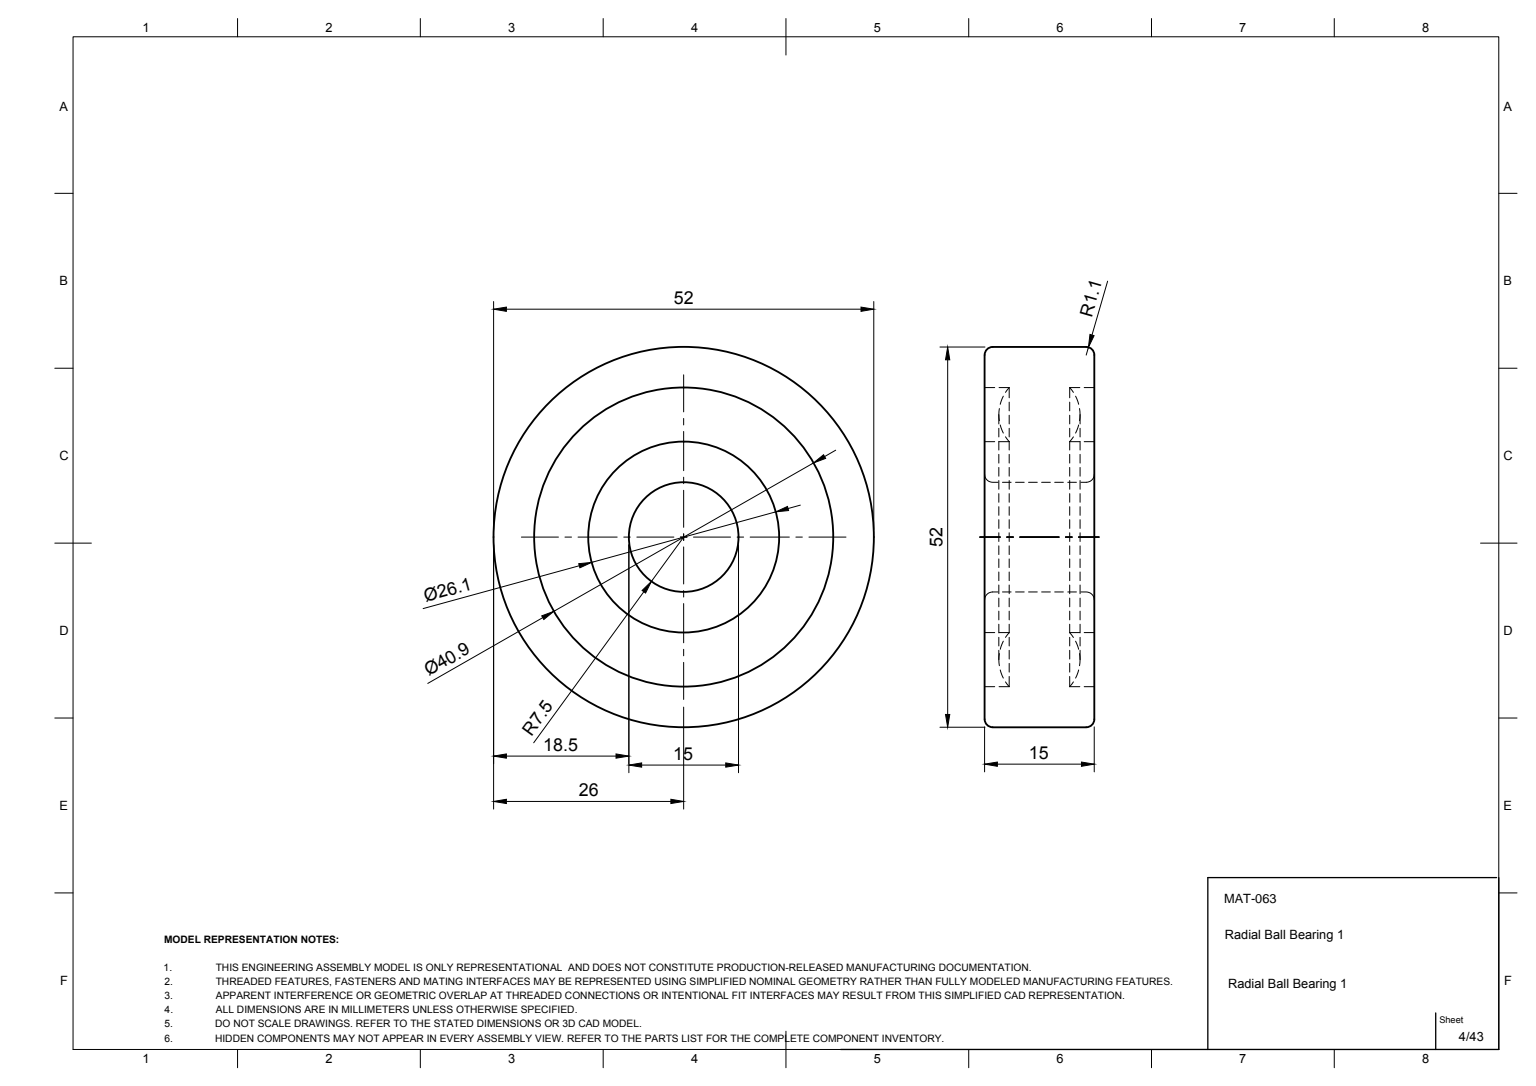
ISO-10303-21;
HEADER;
/* Generated by software containing ST-Developer
 * from STEP Tools, Inc. (www.steptools.com) 
 */

FILE_DESCRIPTION(
/* description */ (''),
/* implementation_level */ '2;1');

FILE_NAME(
/* name */ 'Radial Ball Bearing 1.step',
/* time_stamp */ '2026-10-24T09:43:01-07:00',
/* author */ (''),
/* organization */ (''),
/* preprocessor_version */ 'ST-DEVELOPER v20.2',
/* originating_system */ 'Autodesk Translation Framework v15.15.0.0',
/* authorisation */ '');

FILE_SCHEMA (('AUTOMOTIVE_DESIGN { 1 0 10303 214 3 1 1 }'));
ENDSEC;

DATA;
#10=MECHANICAL_DESIGN_GEOMETRIC_PRESENTATION_REPRESENTATION('',(#274),#11112);
#167=TOROIDAL_SURFACE('',#6462,0.0248999989285722,0.00110000131901909);
#168=TOROIDAL_SURFACE('',#6467,0.0248999989285722,0.00110000131901909);
#169=TOROIDAL_SURFACE('',#6475,0.0248999989285722,0.00110000131901911);
#170=TOROIDAL_SURFACE('',#6482,0.0248999989285722,0.00110000131901911);
#171=TOROIDAL_SURFACE('',#6486,0.01675,0.00555000054498457);
#172=TOROIDAL_SURFACE('',#6495,0.01675,0.00555000054498457);
#173=TOROIDAL_SURFACE('',#6504,0.00860000107142784,0.00110000131901912);
#174=TOROIDAL_SURFACE('',#6508,0.00860000107142784,0.00110000131901912);
#175=TOROIDAL_SURFACE('',#6516,0.00860000107142785,0.00110000131901912);
#176=TOROIDAL_SURFACE('',#6519,0.00860000107142785,0.00110000131901912);
#208=SHAPE_REPRESENTATION_RELATIONSHIP('SRR','None',#11231,#241);
#241=ADVANCED_BREP_SHAPE_REPRESENTATION('',(#307),#11076);
#274=STYLED_ITEM('',(#11425),#307);
#307=MANIFOLD_SOLID_BREP('Radial Ball Bearing 1',#6011);
#357=FACE_BOUND('',#1081,.T.);
#358=FACE_BOUND('',#1086,.T.);
#359=FACE_BOUND('',#1092,.T.);
#360=FACE_BOUND('',#1097,.T.);
#502=PLANE('',#6473);
#503=PLANE('',#6484);
#504=PLANE('',#6499);
#505=PLANE('',#6510);
#695=FACE_OUTER_BOUND('',#1077,.T.);
#696=FACE_OUTER_BOUND('',#1078,.T.);
#697=FACE_OUTER_BOUND('',#1079,.T.);
#698=FACE_OUTER_BOUND('',#1080,.T.);
#699=FACE_OUTER_BOUND('',#1082,.T.);
#700=FACE_OUTER_BOUND('',#1083,.T.);
#701=FACE_OUTER_BOUND('',#1084,.T.);
#702=FACE_OUTER_BOUND('',#1085,.T.);
#703=FACE_OUTER_BOUND('',#1087,.T.);
#704=FACE_OUTER_BOUND('',#1088,.T.);
#705=FACE_OUTER_BOUND('',#1089,.T.);
#706=FACE_OUTER_BOUND('',#1090,.T.);
#707=FACE_OUTER_BOUND('',#1091,.T.);
#708=FACE_OUTER_BOUND('',#1093,.T.);
#709=FACE_OUTER_BOUND('',#1094,.T.);
#710=FACE_OUTER_BOUND('',#1095,.T.);
#711=FACE_OUTER_BOUND('',#1096,.T.);
#712=FACE_OUTER_BOUND('',#1098,.T.);
#713=FACE_OUTER_BOUND('',#1099,.T.);
#714=FACE_OUTER_BOUND('',#1100,.T.);
#1077=EDGE_LOOP('',(#4045,#4046,#4047,#4048));
#1078=EDGE_LOOP('',(#4049,#4050,#4051,#4052));
#1079=EDGE_LOOP('',(#4053,#4054,#4055,#4056,#4057,#4058));
#1080=EDGE_LOOP('',(#4059,#4060));
#1081=EDGE_LOOP('',(#4061));
#1082=EDGE_LOOP('',(#4062,#4063,#4064,#4065));
#1083=EDGE_LOOP('',(#4066,#4067,#4068,#4069,#4070));
#1084=EDGE_LOOP('',(#4071,#4072,#4073,#4074));
#1085=EDGE_LOOP('',(#4075,#4076));
#1086=EDGE_LOOP('',(#4077));
#1087=EDGE_LOOP('',(#4078,#4079,#4080,#4081,#4082,#4083));
#1088=EDGE_LOOP('',(#4084,#4085,#4086,#4087,#4088));
#1089=EDGE_LOOP('',(#4089,#4090,#4091,#4092,#4093));
#1090=EDGE_LOOP('',(#4094,#4095,#4096,#4097,#4098,#4099));
#1091=EDGE_LOOP('',(#4100));
#1092=EDGE_LOOP('',(#4101,#4102));
#1093=EDGE_LOOP('',(#4103,#4104,#4105,#4106,#4107));
#1094=EDGE_LOOP('',(#4108,#4109,#4110,#4111));
#1095=EDGE_LOOP('',(#4112,#4113,#4114,#4115));
#1096=EDGE_LOOP('',(#4116));
#1097=EDGE_LOOP('',(#4117,#4118));
#1098=EDGE_LOOP('',(#4119,#4120,#4121,#4122,#4123,#4124));
#1099=EDGE_LOOP('',(#4125,#4126,#4127,#4128));
#1100=EDGE_LOOP('',(#4129,#4130,#4131,#4132));
#1574=LINE('',#9443,#1933);
#1575=LINE('',#9455,#1934);
#1576=LINE('',#9475,#1935);
#1577=LINE('',#9478,#1936);
#1578=LINE('',#9494,#1937);
#1579=LINE('',#9510,#1938);
#1933=VECTOR('',#7408,0.026);
#1934=VECTOR('',#7423,0.02045);
#1935=VECTOR('',#7450,0.02045);
#1936=VECTOR('',#7453,0.01305);
#1937=VECTOR('',#7474,0.01305);
#1938=VECTOR('',#7495,0.0075);
#2306=CIRCLE('',#6463,0.0248999997701383);
#2307=CIRCLE('',#6464,0.00110000131901909);
#2308=CIRCLE('',#6465,0.0260000002475909);
#2309=CIRCLE('',#6466,0.00110000131901909);
#2310=CIRCLE('',#6468,0.0248999997701383);
#2311=CIRCLE('',#6469,0.0260000002475909);
#2312=CIRCLE('',#6471,0.026);
#2313=CIRCLE('',#6472,0.026);
#2314=CIRCLE('',#6474,0.02045);
#2315=CIRCLE('',#6476,0.00110000131901911);
#2316=CIRCLE('',#6477,0.0248999997701383);
#2317=CIRCLE('',#6478,0.0011000013190191);
#2318=CIRCLE('',#6480,0.02045);
#2319=CIRCLE('',#6481,0.02045);
#2320=CIRCLE('',#6483,0.0248999997701383);
#2321=CIRCLE('',#6485,0.02045);
#2322=CIRCLE('',#6487,0.00555000054498457);
#2323=CIRCLE('',#6488,0.0130499999271107);
#2324=CIRCLE('',#6489,0.0130499999271107);
#2325=CIRCLE('',#6491,0.02045);
#2326=CIRCLE('',#6492,0.02045);
#2327=CIRCLE('',#6494,0.01305);
#2328=CIRCLE('',#6496,0.01305);
#2329=CIRCLE('',#6497,0.00555000054498457);
#2330=CIRCLE('',#6498,0.01305);
#2331=CIRCLE('',#6500,0.00860000022986177);
#2332=CIRCLE('',#6501,0.00860000022986177);
#2333=CIRCLE('',#6503,0.01305);
#2334=CIRCLE('',#6505,0.00110000131901912);
#2335=CIRCLE('',#6506,0.00749999975240907);
#2336=CIRCLE('',#6507,0.00110000131901912);
#2337=CIRCLE('',#6509,0.00749999975240873);
#2338=CIRCLE('',#6511,0.00860000022986177);
#2339=CIRCLE('',#6512,0.00860000022986177);
#2340=CIRCLE('',#6514,0.0075);
#2341=CIRCLE('',#6515,0.00749999975240873);
#2342=CIRCLE('',#6517,0.00110000131901912);
#2343=CIRCLE('',#6518,0.00110000131901912);
#2712=VERTEX_POINT('',#9427);
#2713=VERTEX_POINT('',#9428);
#2714=VERTEX_POINT('',#9430);
#2715=VERTEX_POINT('',#9432);
#2716=VERTEX_POINT('',#9439);
#2717=VERTEX_POINT('',#9440);
#2718=VERTEX_POINT('',#9445);
#2719=VERTEX_POINT('',#9448);
#2720=VERTEX_POINT('',#9450);
#2721=VERTEX_POINT('',#9454);
#2722=VERTEX_POINT('',#9456);
#2723=VERTEX_POINT('',#9462);
#2724=VERTEX_POINT('',#9465);
#2725=VERTEX_POINT('',#9467);
#2726=VERTEX_POINT('',#9471);
#2727=VERTEX_POINT('',#9472);
#2728=VERTEX_POINT('',#9477);
#2729=VERTEX_POINT('',#9481);
#2730=VERTEX_POINT('',#9482);
#2731=VERTEX_POINT('',#9487);
#2732=VERTEX_POINT('',#9488);
#2733=VERTEX_POINT('',#9492);
#2734=VERTEX_POINT('',#9496);
#2735=VERTEX_POINT('',#9498);
#2736=VERTEX_POINT('',#9504);
#2737=VERTEX_POINT('',#9505);
#2738=VERTEX_POINT('',#9509);
#2739=VERTEX_POINT('',#9511);
#3226=EDGE_CURVE('',#2712,#2713,#2306,.T.);
#3227=EDGE_CURVE('',#2713,#2714,#2307,.T.);
#3228=EDGE_CURVE('',#2714,#2715,#2308,.F.);
#3229=EDGE_CURVE('',#2715,#2712,#2309,.T.);
#3230=EDGE_CURVE('',#2713,#2712,#2310,.T.);
#3231=EDGE_CURVE('',#2715,#2714,#2311,.T.);
#3232=EDGE_CURVE('',#2716,#2717,#2312,.F.);
#3233=EDGE_CURVE('',#2717,#2716,#2313,.F.);
#3234=EDGE_CURVE('',#2716,#2714,#1574,.T.);
#3235=EDGE_CURVE('',#2718,#2718,#2314,.T.);
#3236=EDGE_CURVE('',#2716,#2719,#2315,.T.);
#3237=EDGE_CURVE('',#2719,#2720,#2316,.F.);
#3238=EDGE_CURVE('',#2720,#2717,#2317,.T.);
#3239=EDGE_CURVE('',#2718,#2721,#1575,.T.);
#3240=EDGE_CURVE('',#2722,#2721,#2318,.F.);
#3241=EDGE_CURVE('',#2721,#2722,#2319,.F.);
#3242=EDGE_CURVE('',#2720,#2719,#2320,.F.);
#3243=EDGE_CURVE('',#2723,#2723,#2321,.F.);
#3244=EDGE_CURVE('',#2722,#2724,#2322,.T.);
#3245=EDGE_CURVE('',#2724,#2725,#2323,.T.);
#3246=EDGE_CURVE('',#2725,#2724,#2324,.T.);
#3247=EDGE_CURVE('',#2726,#2727,#2325,.F.);
#3248=EDGE_CURVE('',#2727,#2726,#2326,.F.);
#3249=EDGE_CURVE('',#2727,#2723,#1576,.T.);
#3250=EDGE_CURVE('',#2725,#2728,#1577,.T.);
#3251=EDGE_CURVE('',#2728,#2728,#2327,.T.);
#3252=EDGE_CURVE('',#2729,#2730,#2328,.T.);
#3253=EDGE_CURVE('',#2730,#2726,#2329,.T.);
#3254=EDGE_CURVE('',#2730,#2729,#2330,.T.);
#3255=EDGE_CURVE('',#2731,#2732,#2331,.T.);
#3256=EDGE_CURVE('',#2732,#2731,#2332,.T.);
#3257=EDGE_CURVE('',#2733,#2733,#2333,.F.);
#3258=EDGE_CURVE('',#2733,#2729,#1578,.T.);
#3259=EDGE_CURVE('',#2732,#2734,#2334,.T.);
#3260=EDGE_CURVE('',#2734,#2735,#2335,.T.);
#3261=EDGE_CURVE('',#2735,#2731,#2336,.T.);
#3262=EDGE_CURVE('',#2735,#2734,#2337,.T.);
#3263=EDGE_CURVE('',#2736,#2737,#2338,.F.);
#3264=EDGE_CURVE('',#2737,#2736,#2339,.F.);
#3265=EDGE_CURVE('',#2734,#2738,#1579,.T.);
#3266=EDGE_CURVE('',#2739,#2738,#2340,.F.);
#3267=EDGE_CURVE('',#2738,#2739,#2341,.F.);
#3268=EDGE_CURVE('',#2738,#2736,#2342,.T.);
#3269=EDGE_CURVE('',#2737,#2739,#2343,.T.);
#4045=ORIENTED_EDGE('',*,*,#3226,.T.);
#4046=ORIENTED_EDGE('',*,*,#3227,.T.);
#4047=ORIENTED_EDGE('',*,*,#3228,.T.);
#4048=ORIENTED_EDGE('',*,*,#3229,.T.);
#4049=ORIENTED_EDGE('',*,*,#3227,.F.);
#4050=ORIENTED_EDGE('',*,*,#3230,.T.);
#4051=ORIENTED_EDGE('',*,*,#3229,.F.);
#4052=ORIENTED_EDGE('',*,*,#3231,.T.);
#4053=ORIENTED_EDGE('',*,*,#3232,.T.);
#4054=ORIENTED_EDGE('',*,*,#3233,.T.);
#4055=ORIENTED_EDGE('',*,*,#3234,.T.);
#4056=ORIENTED_EDGE('',*,*,#3231,.F.);
#4057=ORIENTED_EDGE('',*,*,#3228,.F.);
#4058=ORIENTED_EDGE('',*,*,#3234,.F.);
#4059=ORIENTED_EDGE('',*,*,#3226,.F.);
#4060=ORIENTED_EDGE('',*,*,#3230,.F.);
#4061=ORIENTED_EDGE('',*,*,#3235,.T.);
#4062=ORIENTED_EDGE('',*,*,#3232,.F.);
#4063=ORIENTED_EDGE('',*,*,#3236,.T.);
#4064=ORIENTED_EDGE('',*,*,#3237,.T.);
#4065=ORIENTED_EDGE('',*,*,#3238,.T.);
#4066=ORIENTED_EDGE('',*,*,#3235,.F.);
#4067=ORIENTED_EDGE('',*,*,#3239,.T.);
#4068=ORIENTED_EDGE('',*,*,#3240,.F.);
#4069=ORIENTED_EDGE('',*,*,#3241,.F.);
#4070=ORIENTED_EDGE('',*,*,#3239,.F.);
#4071=ORIENTED_EDGE('',*,*,#3236,.F.);
#4072=ORIENTED_EDGE('',*,*,#3233,.F.);
#4073=ORIENTED_EDGE('',*,*,#3238,.F.);
#4074=ORIENTED_EDGE('',*,*,#3242,.T.);
#4075=ORIENTED_EDGE('',*,*,#3237,.F.);
#4076=ORIENTED_EDGE('',*,*,#3242,.F.);
#4077=ORIENTED_EDGE('',*,*,#3243,.T.);
#4078=ORIENTED_EDGE('',*,*,#3241,.T.);
#4079=ORIENTED_EDGE('',*,*,#3244,.T.);
#4080=ORIENTED_EDGE('',*,*,#3245,.T.);
#4081=ORIENTED_EDGE('',*,*,#3246,.T.);
#4082=ORIENTED_EDGE('',*,*,#3244,.F.);
#4083=ORIENTED_EDGE('',*,*,#3240,.T.);
#4084=ORIENTED_EDGE('',*,*,#3247,.F.);
#4085=ORIENTED_EDGE('',*,*,#3248,.F.);
#4086=ORIENTED_EDGE('',*,*,#3249,.T.);
#4087=ORIENTED_EDGE('',*,*,#3243,.F.);
#4088=ORIENTED_EDGE('',*,*,#3249,.F.);
#4089=ORIENTED_EDGE('',*,*,#3246,.F.);
#4090=ORIENTED_EDGE('',*,*,#3250,.T.);
#4091=ORIENTED_EDGE('',*,*,#3251,.T.);
#4092=ORIENTED_EDGE('',*,*,#3250,.F.);
#4093=ORIENTED_EDGE('',*,*,#3245,.F.);
#4094=ORIENTED_EDGE('',*,*,#3252,.T.);
#4095=ORIENTED_EDGE('',*,*,#3253,.T.);
#4096=ORIENTED_EDGE('',*,*,#3247,.T.);
#4097=ORIENTED_EDGE('',*,*,#3248,.T.);
#4098=ORIENTED_EDGE('',*,*,#3253,.F.);
#4099=ORIENTED_EDGE('',*,*,#3254,.T.);
#4100=ORIENTED_EDGE('',*,*,#3251,.F.);
#4101=ORIENTED_EDGE('',*,*,#3255,.T.);
#4102=ORIENTED_EDGE('',*,*,#3256,.T.);
#4103=ORIENTED_EDGE('',*,*,#3257,.T.);
#4104=ORIENTED_EDGE('',*,*,#3258,.T.);
#4105=ORIENTED_EDGE('',*,*,#3254,.F.);
#4106=ORIENTED_EDGE('',*,*,#3252,.F.);
#4107=ORIENTED_EDGE('',*,*,#3258,.F.);
#4108=ORIENTED_EDGE('',*,*,#3259,.T.);
#4109=ORIENTED_EDGE('',*,*,#3260,.T.);
#4110=ORIENTED_EDGE('',*,*,#3261,.T.);
#4111=ORIENTED_EDGE('',*,*,#3256,.F.);
#4112=ORIENTED_EDGE('',*,*,#3262,.T.);
#4113=ORIENTED_EDGE('',*,*,#3259,.F.);
#4114=ORIENTED_EDGE('',*,*,#3255,.F.);
#4115=ORIENTED_EDGE('',*,*,#3261,.F.);
#4116=ORIENTED_EDGE('',*,*,#3257,.F.);
#4117=ORIENTED_EDGE('',*,*,#3263,.T.);
#4118=ORIENTED_EDGE('',*,*,#3264,.T.);
#4119=ORIENTED_EDGE('',*,*,#3260,.F.);
#4120=ORIENTED_EDGE('',*,*,#3265,.T.);
#4121=ORIENTED_EDGE('',*,*,#3266,.F.);
#4122=ORIENTED_EDGE('',*,*,#3267,.F.);
#4123=ORIENTED_EDGE('',*,*,#3265,.F.);
#4124=ORIENTED_EDGE('',*,*,#3262,.F.);
#4125=ORIENTED_EDGE('',*,*,#3268,.T.);
#4126=ORIENTED_EDGE('',*,*,#3264,.F.);
#4127=ORIENTED_EDGE('',*,*,#3269,.T.);
#4128=ORIENTED_EDGE('',*,*,#3266,.T.);
#4129=ORIENTED_EDGE('',*,*,#3263,.F.);
#4130=ORIENTED_EDGE('',*,*,#3268,.F.);
#4131=ORIENTED_EDGE('',*,*,#3267,.T.);
#4132=ORIENTED_EDGE('',*,*,#3269,.F.);
#5513=CYLINDRICAL_SURFACE('',#6470,0.026);
#5514=CYLINDRICAL_SURFACE('',#6479,0.02045);
#5515=CYLINDRICAL_SURFACE('',#6490,0.02045);
#5516=CYLINDRICAL_SURFACE('',#6493,0.01305);
#5517=CYLINDRICAL_SURFACE('',#6502,0.01305);
#5518=CYLINDRICAL_SURFACE('',#6513,0.0075);
#5668=ADVANCED_FACE('',(#695),#167,.T.);
#5669=ADVANCED_FACE('',(#696),#168,.T.);
#5670=ADVANCED_FACE('',(#697),#5513,.T.);
#5671=ADVANCED_FACE('',(#698,#357),#502,.T.);
#5672=ADVANCED_FACE('',(#699),#169,.T.);
#5673=ADVANCED_FACE('',(#700),#5514,.F.);
#5674=ADVANCED_FACE('',(#701),#170,.T.);
#5675=ADVANCED_FACE('',(#702,#358),#503,.T.);
#5676=ADVANCED_FACE('',(#703),#171,.T.);
#5677=ADVANCED_FACE('',(#704),#5515,.F.);
#5678=ADVANCED_FACE('',(#705),#5516,.T.);
#5679=ADVANCED_FACE('',(#706),#172,.T.);
#5680=ADVANCED_FACE('',(#707,#359),#504,.T.);
#5681=ADVANCED_FACE('',(#708),#5517,.T.);
#5682=ADVANCED_FACE('',(#709),#173,.T.);
#5683=ADVANCED_FACE('',(#710),#174,.T.);
#5684=ADVANCED_FACE('',(#711,#360),#505,.T.);
#5685=ADVANCED_FACE('',(#712),#5518,.F.);
#5686=ADVANCED_FACE('',(#713),#175,.T.);
#5687=ADVANCED_FACE('',(#714),#176,.T.);
#6011=CLOSED_SHELL('',(#5668,#5669,#5670,#5671,#5672,#5673,#5674,#5675,
#5676,#5677,#5678,#5679,#5680,#5681,#5682,#5683,#5684,#5685,#5686,#5687));
#6461=AXIS2_PLACEMENT_3D('',#9425,#7384,#7385);
#6462=AXIS2_PLACEMENT_3D('',#9426,#7386,#7387);
#6463=AXIS2_PLACEMENT_3D('',#9429,#7388,#7389);
#6464=AXIS2_PLACEMENT_3D('',#9431,#7390,#7391);
#6465=AXIS2_PLACEMENT_3D('',#9433,#7392,#7393);
#6466=AXIS2_PLACEMENT_3D('',#9434,#7394,#7395);
#6467=AXIS2_PLACEMENT_3D('',#9435,#7396,#7397);
#6468=AXIS2_PLACEMENT_3D('',#9436,#7398,#7399);
#6469=AXIS2_PLACEMENT_3D('',#9437,#7400,#7401);
#6470=AXIS2_PLACEMENT_3D('',#9438,#7402,#7403);
#6471=AXIS2_PLACEMENT_3D('',#9441,#7404,#7405);
#6472=AXIS2_PLACEMENT_3D('',#9442,#7406,#7407);
#6473=AXIS2_PLACEMENT_3D('',#9444,#7409,#7410);
#6474=AXIS2_PLACEMENT_3D('',#9446,#7411,#7412);
#6475=AXIS2_PLACEMENT_3D('',#9447,#7413,#7414);
#6476=AXIS2_PLACEMENT_3D('',#9449,#7415,#7416);
#6477=AXIS2_PLACEMENT_3D('',#9451,#7417,#7418);
#6478=AXIS2_PLACEMENT_3D('',#9452,#7419,#7420);
#6479=AXIS2_PLACEMENT_3D('',#9453,#7421,#7422);
#6480=AXIS2_PLACEMENT_3D('',#9457,#7424,#7425);
#6481=AXIS2_PLACEMENT_3D('',#9458,#7426,#7427);
#6482=AXIS2_PLACEMENT_3D('',#9459,#7428,#7429);
#6483=AXIS2_PLACEMENT_3D('',#9460,#7430,#7431);
#6484=AXIS2_PLACEMENT_3D('',#9461,#7432,#7433);
#6485=AXIS2_PLACEMENT_3D('',#9463,#7434,#7435);
#6486=AXIS2_PLACEMENT_3D('',#9464,#7436,#7437);
#6487=AXIS2_PLACEMENT_3D('',#9466,#7438,#7439);
#6488=AXIS2_PLACEMENT_3D('',#9468,#7440,#7441);
#6489=AXIS2_PLACEMENT_3D('',#9469,#7442,#7443);
#6490=AXIS2_PLACEMENT_3D('',#9470,#7444,#7445);
#6491=AXIS2_PLACEMENT_3D('',#9473,#7446,#7447);
#6492=AXIS2_PLACEMENT_3D('',#9474,#7448,#7449);
#6493=AXIS2_PLACEMENT_3D('',#9476,#7451,#7452);
#6494=AXIS2_PLACEMENT_3D('',#9479,#7454,#7455);
#6495=AXIS2_PLACEMENT_3D('',#9480,#7456,#7457);
#6496=AXIS2_PLACEMENT_3D('',#9483,#7458,#7459);
#6497=AXIS2_PLACEMENT_3D('',#9484,#7460,#7461);
#6498=AXIS2_PLACEMENT_3D('',#9485,#7462,#7463);
#6499=AXIS2_PLACEMENT_3D('',#9486,#7464,#7465);
#6500=AXIS2_PLACEMENT_3D('',#9489,#7466,#7467);
#6501=AXIS2_PLACEMENT_3D('',#9490,#7468,#7469);
#6502=AXIS2_PLACEMENT_3D('',#9491,#7470,#7471);
#6503=AXIS2_PLACEMENT_3D('',#9493,#7472,#7473);
#6504=AXIS2_PLACEMENT_3D('',#9495,#7475,#7476);
#6505=AXIS2_PLACEMENT_3D('',#9497,#7477,#7478);
#6506=AXIS2_PLACEMENT_3D('',#9499,#7479,#7480);
#6507=AXIS2_PLACEMENT_3D('',#9500,#7481,#7482);
#6508=AXIS2_PLACEMENT_3D('',#9501,#7483,#7484);
#6509=AXIS2_PLACEMENT_3D('',#9502,#7485,#7486);
#6510=AXIS2_PLACEMENT_3D('',#9503,#7487,#7488);
#6511=AXIS2_PLACEMENT_3D('',#9506,#7489,#7490);
#6512=AXIS2_PLACEMENT_3D('',#9507,#7491,#7492);
#6513=AXIS2_PLACEMENT_3D('',#9508,#7493,#7494);
#6514=AXIS2_PLACEMENT_3D('',#9512,#7496,#7497);
#6515=AXIS2_PLACEMENT_3D('',#9513,#7498,#7499);
#6516=AXIS2_PLACEMENT_3D('',#9514,#7500,#7501);
#6517=AXIS2_PLACEMENT_3D('',#9515,#7502,#7503);
#6518=AXIS2_PLACEMENT_3D('',#9516,#7504,#7505);
#6519=AXIS2_PLACEMENT_3D('',#9517,#7506,#7507);
#7384=DIRECTION('axis',(0.,0.,1.));
#7385=DIRECTION('refdir',(1.,0.,0.));
#7386=DIRECTION('center_axis',(1.,4.17203717831812E-9,1.01277540341552E-17));
#7387=DIRECTION('ref_axis',(-4.1720371751696E-9,1.,0.));
#7388=DIRECTION('center_axis',(1.,4.17203717831812E-9,1.01277540341552E-17));
#7389=DIRECTION('ref_axis',(-4.17203717831812E-9,1.,-1.69634196247466E-42));
#7390=DIRECTION('center_axis',(8.36866394062756E-10,1.,-8.36884415538179E-10));
#7391=DIRECTION('ref_axis',(-7.96162761077703E-7,8.36885081819775E-10,0.999999999999683));
#7392=DIRECTION('center_axis',(1.,4.17203717831812E-9,1.01277540341552E-17));
#7393=DIRECTION('ref_axis',(-4.17203717831812E-9,1.,-1.69634196247466E-42));
#7394=DIRECTION('center_axis',(8.36869948186391E-10,1.,8.36891441629708E-10));
#7395=DIRECTION('ref_axis',(-0.999999999999707,8.36870588457614E-10,-7.65059166582913E-7));
#7396=DIRECTION('center_axis',(1.,-4.17203708245403E-9,6.73890284431642E-18));
#7397=DIRECTION('ref_axis',(-4.1720370750894E-9,-1.,5.66553889764798E-16));
#7398=DIRECTION('center_axis',(1.,-4.17203708245403E-9,6.73890284431642E-18));
#7399=DIRECTION('ref_axis',(4.17203708245403E-9,1.,-1.23465054354127E-43));
#7400=DIRECTION('center_axis',(-1.,4.17203697154146E-9,4.27849718847752E-19));
#7401=DIRECTION('ref_axis',(-4.27008851558771E-17,-5.34839554841822E-9,
1.));
#7402=DIRECTION('center_axis',(1.,0.,-3.33600668457079E-17));
#7403=DIRECTION('ref_axis',(-3.33600668457079E-17,0.,-1.));
#7404=DIRECTION('center_axis',(1.,0.,-3.33600668457079E-17));
#7405=DIRECTION('ref_axis',(-3.33600668457079E-17,0.,-1.));
#7406=DIRECTION('center_axis',(1.,0.,0.));
#7407=DIRECTION('ref_axis',(0.,-4.64793894161955E-10,-1.));
#7408=DIRECTION('',(-1.,0.,3.33600668457079E-17));
#7409=DIRECTION('center_axis',(-1.,1.53144334479515E-17,1.9842828066192E-17));
#7410=DIRECTION('ref_axis',(1.9842828066192E-17,0.,1.));
#7411=DIRECTION('center_axis',(1.,0.,0.));
#7412=DIRECTION('ref_axis',(0.,0.,-1.));
#7413=DIRECTION('center_axis',(1.,-4.17203727418451E-9,-1.07069540457721E-17));
#7414=DIRECTION('ref_axis',(4.1720372752498E-9,1.,0.));
#7415=DIRECTION('center_axis',(-8.36866342496331E-10,1.,-8.36883936494317E-10));
#7416=DIRECTION('ref_axis',(0.999999999999707,8.36866982761818E-10,7.65059174657239E-7));
#7417=DIRECTION('center_axis',(1.,-4.17203727418451E-9,-1.07069540457721E-17));
#7418=DIRECTION('ref_axis',(4.17203727418451E-9,1.,1.45967462857766E-42));
#7419=DIRECTION('center_axis',(-8.36844869453255E-10,1.,8.36865935422119E-10));
#7420=DIRECTION('ref_axis',(9.00645352209864E-7,8.36866689122222E-10,-0.999999999999595));
#7421=DIRECTION('center_axis',(1.,0.,0.));
#7422=DIRECTION('ref_axis',(0.,0.,-1.));
#7423=DIRECTION('',(1.,0.,0.));
#7424=DIRECTION('center_axis',(1.,0.,0.));
#7425=DIRECTION('ref_axis',(0.,-4.29586394988857E-10,-1.));
#7426=DIRECTION('center_axis',(1.,0.,0.));
#7427=DIRECTION('ref_axis',(0.,-4.29586394988857E-10,-1.));
#7428=DIRECTION('center_axis',(1.,4.17203725971588E-9,2.0031116033889E-18));
#7429=DIRECTION('ref_axis',(4.1720372752498E-9,-1.,5.66553889764798E-16));
#7430=DIRECTION('center_axis',(1.,4.17203725971588E-9,2.0031116033889E-18));
#7431=DIRECTION('ref_axis',(-4.17203725971588E-9,1.,5.39459847610519E-43));
#7432=DIRECTION('center_axis',(1.,1.53144334479515E-17,-1.9842828066192E-17));
#7433=DIRECTION('ref_axis',(-1.9842828066192E-17,0.,-1.));
#7434=DIRECTION('center_axis',(1.,0.,0.));
#7435=DIRECTION('ref_axis',(0.,0.,-1.));
#7436=DIRECTION('center_axis',(1.,6.36556116938371E-17,1.00386354793954E-17));
#7437=DIRECTION('ref_axis',(-6.3655612933414E-17,1.,0.));
#7438=DIRECTION('center_axis',(1.00386354793954E-17,1.22464679914735E-16,
-1.));
#7439=DIRECTION('ref_axis',(6.36556105223495E-17,-1.,-1.22464679914735E-16));
#7440=DIRECTION('center_axis',(1.,1.35504238326755E-16,2.34999225611352E-17));
#7441=DIRECTION('ref_axis',(-1.35504238326755E-16,1.,1.40763492406121E-49));
#7442=DIRECTION('center_axis',(1.,1.35504238326755E-16,2.34999225611352E-17));
#7443=DIRECTION('ref_axis',(-1.35504238326755E-16,1.,1.40763492406121E-49));
#7444=DIRECTION('center_axis',(1.,0.,0.));
#7445=DIRECTION('ref_axis',(0.,0.,-1.));
#7446=DIRECTION('center_axis',(-1.,0.,0.));
#7447=DIRECTION('ref_axis',(0.,-6.60206605267583E-10,1.));
#7448=DIRECTION('center_axis',(-1.,0.,0.));
#7449=DIRECTION('ref_axis',(0.,-6.60206605267583E-10,1.));
#7450=DIRECTION('',(1.,0.,0.));
#7451=DIRECTION('center_axis',(1.,0.,0.));
#7452=DIRECTION('ref_axis',(0.,0.,-1.));
#7453=DIRECTION('',(-1.,0.,0.));
#7454=DIRECTION('center_axis',(1.,0.,0.));
#7455=DIRECTION('ref_axis',(0.,0.,-1.));
#7456=DIRECTION('center_axis',(1.,1.18552772674719E-16,-1.97711088800387E-17));
#7457=DIRECTION('ref_axis',(-1.18552772074394E-16,1.,0.));
#7458=DIRECTION('center_axis',(-1.,0.,0.));
#7459=DIRECTION('ref_axis',(0.,-2.05103586755523E-10,1.));
#7460=DIRECTION('center_axis',(-1.97711088800387E-17,1.22464679914735E-16,
-1.));
#7461=DIRECTION('ref_axis',(1.18552771796194E-16,-1.,-1.22464679914735E-16));
#7462=DIRECTION('center_axis',(-1.,0.,0.));
#7463=DIRECTION('ref_axis',(0.,-2.05103586755523E-10,1.));
#7464=DIRECTION('center_axis',(-1.,2.92206431305708E-17,3.78610282642285E-17));
#7465=DIRECTION('ref_axis',(3.78610282642285E-17,0.,1.));
#7466=DIRECTION('center_axis',(1.,1.20795004338275E-8,6.525328094131E-17));
#7467=DIRECTION('ref_axis',(-1.20795004338275E-8,1.,4.44135209129409E-41));
#7468=DIRECTION('center_axis',(1.,-1.20794999078492E-8,-6.65136044666218E-17));
#7469=DIRECTION('ref_axis',(1.20794999078492E-8,1.,-3.20659696454606E-41));
#7470=DIRECTION('center_axis',(1.,0.,0.));
#7471=DIRECTION('ref_axis',(0.,0.,-1.));
#7472=DIRECTION('center_axis',(1.,0.,0.));
#7473=DIRECTION('ref_axis',(0.,0.,-1.));
#7474=DIRECTION('',(-1.,0.,0.));
#7475=DIRECTION('center_axis',(1.,-1.20794999078492E-8,-6.65136044666218E-17));
#7476=DIRECTION('ref_axis',(-1.20794999243885E-8,-1.,-5.21792575105832E-12));
#7477=DIRECTION('center_axis',(-3.90112644891662E-10,-1.,-3.90117034748036E-10));
#7478=DIRECTION('ref_axis',(-7.96162782272821E-7,3.90117345341081E-10,-0.999999999999683));
#7479=DIRECTION('center_axis',(1.,-1.20794992145421E-8,-4.8381018443521E-19));
#7480=DIRECTION('ref_axis',(1.48029741503464E-16,1.78300800621899E-8,-1.));
#7481=DIRECTION('center_axis',(-3.90083830404282E-10,-1.,3.90119162273478E-10));
#7482=DIRECTION('ref_axis',(-0.999999999999707,3.90084128868405E-10,7.65059156489968E-7));
#7483=DIRECTION('center_axis',(1.,1.20795004338275E-8,6.525328094131E-17));
#7484=DIRECTION('ref_axis',(-1.20795004609008E-8,1.,0.));
#7485=DIRECTION('center_axis',(1.,1.20795004338275E-8,6.525328094131E-17));
#7486=DIRECTION('ref_axis',(-1.20795004338275E-8,1.,4.44135209129409E-41));
#7487=DIRECTION('center_axis',(1.,2.92206431305708E-17,-3.78610282642285E-17));
#7488=DIRECTION('ref_axis',(-3.78610282642285E-17,0.,-1.));
#7489=DIRECTION('center_axis',(1.,-1.20794999071527E-8,2.28224857621035E-17));
#7490=DIRECTION('ref_axis',(1.20794999071527E-8,1.,-1.89856639006012E-41));
#7491=DIRECTION('center_axis',(1.,1.20794999172425E-8,-1.59545740616835E-17));
#7492=DIRECTION('ref_axis',(-1.20794999172425E-8,1.,2.99570552288603E-42));
#7493=DIRECTION('center_axis',(1.,0.,-1.15648231731787E-16));
#7494=DIRECTION('ref_axis',(-1.15648231731787E-16,0.,-1.));
#7495=DIRECTION('',(1.,0.,-1.15648231731787E-16));
#7496=DIRECTION('center_axis',(1.,0.,0.));
#7497=DIRECTION('ref_axis',(0.,-4.29586131949163E-10,-1.));
#7498=DIRECTION('center_axis',(1.,-1.20794999071527E-8,2.28224857621035E-17));
#7499=DIRECTION('ref_axis',(1.20794999071527E-8,1.,-1.89856639006012E-41));
#7500=DIRECTION('center_axis',(1.,1.20794999172425E-8,-1.59545740616835E-17));
#7501=DIRECTION('ref_axis',(1.20794999243885E-8,-1.,-8.2319592183107E-12));
#7502=DIRECTION('center_axis',(3.9010897446429E-10,-1.,-3.90108144056802E-10));
#7503=DIRECTION('ref_axis',(0.999999999999707,3.90109272919983E-10,-7.65059154471383E-7));
#7504=DIRECTION('center_axis',(3.90083837031876E-10,-1.,3.90119162425402E-10));
#7505=DIRECTION('ref_axis',(7.96162783282112E-7,3.90119472995512E-10,0.999999999999683));
#7506=DIRECTION('center_axis',(1.,-1.20794999071527E-8,2.28224857621035E-17));
#7507=DIRECTION('ref_axis',(1.20794999243885E-8,1.,0.));
#9425=CARTESIAN_POINT('',(0.,0.,0.));
#9426=CARTESIAN_POINT('Origin',(-0.00639999889435817,-1.33725586897056E-10,
-2.60202312123977E-18));
#9427=CARTESIAN_POINT('',(-0.00750000021337694,-2.62982038223811E-17,-0.0248999997701383));
#9428=CARTESIAN_POINT('',(-0.00750000021337694,-9.33158505355009E-18,0.0248999997701383));
#9429=CARTESIAN_POINT('Origin',(-0.00750000021337694,-1.38314833296201E-10,
-2.61316366403604E-18));
#9430=CARTESIAN_POINT('',(-0.00639999976976533,-1.58005919577827E-12,0.0260000002475909));
#9431=CARTESIAN_POINT('Origin',(-0.00639999889435817,-9.20581548326642E-13,
0.0248999989285722));
#9432=CARTESIAN_POINT('',(-0.00639999976976533,-3.35121902792442E-17,-0.0260000002475909));
#9433=CARTESIAN_POINT('Origin',(-0.00639999977013826,-1.33725590550843E-10,
-2.60202313010945E-18));
#9434=CARTESIAN_POINT('Origin',(-0.00639999889435817,-9.20629689158185E-13,
-0.0248999989285722));
#9435=CARTESIAN_POINT('Origin',(-0.00639999889435817,1.33725588194013E-10,
-2.25687613815873E-19));
#9436=CARTESIAN_POINT('Origin',(-0.00750000021337694,1.38314834487708E-10,
-2.3310041583336E-19));
#9437=CARTESIAN_POINT('Origin',(-0.00639999977013826,1.3372558821988E-10,
4.44089209850063E-18));
#9438=CARTESIAN_POINT('Origin',(-0.0206375,0.,-4.33144407778805E-52));
#9439=CARTESIAN_POINT('',(0.00639999998722997,-6.70342338705283E-12,0.0260000000825303));
#9440=CARTESIAN_POINT('',(0.00639999998722997,-5.37097589710219E-12,-0.0260000000825303));
#9441=CARTESIAN_POINT('Origin',(0.0064,0.,-9.01972807340825E-19));
#9442=CARTESIAN_POINT('Origin',(0.0064,2.91826343292479E-18,0.));
#9443=CARTESIAN_POINT('',(-0.0206375,-3.18408167778312E-18,0.026));
#9444=CARTESIAN_POINT('Origin',(-0.0075,-1.31838984174237E-18,-1.2490009027033E-18));
#9445=CARTESIAN_POINT('',(-0.0075,-2.50440270425634E-18,0.02045));
#9446=CARTESIAN_POINT('Origin',(-0.0075,0.,0.));
#9447=CARTESIAN_POINT('Origin',(0.00639999889435816,-1.33725593635445E-10,
-3.59711256079879E-19));
#9448=CARTESIAN_POINT('',(0.00750000021337694,-1.05191955076574E-17,0.0248999997701383));
#9449=CARTESIAN_POINT('Origin',(0.00639999889435816,-9.20588335445364E-13,
0.0248999989285722));
#9450=CARTESIAN_POINT('',(0.00750000021337694,-2.93287844693988E-17,-0.0248999997701383));
#9451=CARTESIAN_POINT('Origin',(0.00750000021337694,-1.38314840140043E-10,
-3.71488919652902E-19));
#9452=CARTESIAN_POINT('Origin',(0.00639999889435816,-9.20608946339399E-13,
-0.0248999989285722));
#9453=CARTESIAN_POINT('Origin',(-0.0206375,0.,0.));
#9454=CARTESIAN_POINT('',(-0.00413672599961696,1.0458235455062E-18,0.0204500000364447));
#9455=CARTESIAN_POINT('',(-0.0206375,-2.50440270425634E-18,0.02045));
#9456=CARTESIAN_POINT('',(-0.004136726,-0.02045,-2.79956704802153E-18));
#9457=CARTESIAN_POINT('Origin',(-0.004136726,1.15025496390116E-19,8.88178419700125E-18));
#9458=CARTESIAN_POINT('Origin',(-0.004136726,1.15025496390116E-19,8.88178419700125E-18));
#9459=CARTESIAN_POINT('Origin',(0.00639999889435816,1.33725592594967E-10,
2.43522299685913E-19));
#9460=CARTESIAN_POINT('Origin',(0.00750000021337694,1.3831483908365E-10,
2.45725725091783E-19));
#9461=CARTESIAN_POINT('Origin',(0.0075,-1.31838984174237E-18,1.2490009027033E-18));
#9462=CARTESIAN_POINT('',(0.0075,-2.50440270425634E-18,0.02045));
#9463=CARTESIAN_POINT('Origin',(0.0075,0.,0.));
#9464=CARTESIAN_POINT('Origin',(4.25120033285821E-10,2.32696931299848E-18,
-2.53637255105429E-19));
#9465=CARTESIAN_POINT('',(-0.00413672599923392,-0.0130499999271107,-1.89332840771843E-18));
#9466=CARTESIAN_POINT('Origin',(4.25120034352053E-10,-0.01675,-2.30492064367725E-18));
#9467=CARTESIAN_POINT('',(-0.00413672599923392,-9.72427111671565E-12,0.0130499999635554));
#9468=CARTESIAN_POINT('Origin',(-0.00413672599923392,-2.48296911984889E-18,
-8.56610574398074E-20));
#9469=CARTESIAN_POINT('Origin',(-0.00413672599923392,-2.48296911984889E-18,
-8.56610574398074E-20));
#9470=CARTESIAN_POINT('Origin',(-0.0206375,0.,0.));
#9471=CARTESIAN_POINT('',(0.004136726,-0.02045,-1.97855791081413E-18));
#9472=CARTESIAN_POINT('',(0.004136726,-2.50440270425634E-18,0.02045));
#9473=CARTESIAN_POINT('Origin',(0.004136726,-1.49874617044541E-18,-8.88178419700125E-18));
#9474=CARTESIAN_POINT('Origin',(0.004136726,-1.49874617044541E-18,-8.88178419700125E-18));
#9475=CARTESIAN_POINT('',(-0.0206375,-2.50440270425634E-18,0.02045));
#9476=CARTESIAN_POINT('Origin',(-0.0206375,0.,0.));
#9477=CARTESIAN_POINT('',(-0.0075,-1.5981640728873E-18,0.01305));
#9478=CARTESIAN_POINT('',(-0.0206375,-1.5981640728873E-18,0.01305));
#9479=CARTESIAN_POINT('Origin',(-0.0075,0.,0.));
#9480=CARTESIAN_POINT('Origin',(-4.25120036303284E-10,3.75386134271222E-18,
6.07632462000188E-19));
#9481=CARTESIAN_POINT('',(0.00413672599923392,-2.67659699192252E-12,0.0130499999635553));
#9482=CARTESIAN_POINT('',(0.00413672599923392,-0.01305,-1.07231927942994E-18));
#9483=CARTESIAN_POINT('Origin',(0.00413672599923392,-3.3221160294436E-19,
2.22044604925031E-18));
#9484=CARTESIAN_POINT('Origin',(-4.25120034317525E-10,-0.01675,-1.44365092657163E-18));
#9485=CARTESIAN_POINT('Origin',(0.00413672599923392,-3.3221160294436E-19,
2.22044604925031E-18));
#9486=CARTESIAN_POINT('Origin',(-0.0075,-1.3010426069826E-19,-1.1666015375944E-18));
#9487=CARTESIAN_POINT('',(-0.00750000021337695,-7.32444758467801E-18,-0.00860000022986174));
#9488=CARTESIAN_POINT('',(-0.00750000021337695,-9.55563692214474E-13,0.00860000022983698));
#9489=CARTESIAN_POINT('Origin',(-0.00750000021337695,1.20438122996688E-10,
1.91155415755433E-19));
#9490=CARTESIAN_POINT('Origin',(-0.00750000021337695,-1.20438124044286E-10,
-1.263242268E-19));
#9491=CARTESIAN_POINT('Origin',(-0.0206375,0.,0.));
#9492=CARTESIAN_POINT('',(0.0075,-1.5981640728873E-18,0.01305));
#9493=CARTESIAN_POINT('Origin',(0.0075,0.,0.));
#9494=CARTESIAN_POINT('',(-0.0206375,-1.5981640728873E-18,0.01305));
#9495=CARTESIAN_POINT('Origin',(-0.00639999889435815,-1.33725589876008E-10,
-1.99489279445979E-19));
#9496=CARTESIAN_POINT('',(-0.00639999933187528,-1.78004529143068E-13,0.00749999975240887));
#9497=CARTESIAN_POINT('Origin',(-0.00639999889435815,-4.29138899262724E-13,
0.00860000107142784));
#9498=CARTESIAN_POINT('',(-0.00639999933187528,7.82593383085413E-14,-0.00749999975240887));
#9499=CARTESIAN_POINT('Origin',(-0.00639999977013826,-1.33725577217623E-10,
-2.22044604925031E-18));
#9500=CARTESIAN_POINT('Origin',(-0.00639999889435815,-4.29112928832131E-13,
-0.00860000107142784));
#9501=CARTESIAN_POINT('Origin',(-0.00639999889435816,1.33725589406987E-10,
2.62934110861178E-19));
#9502=CARTESIAN_POINT('Origin',(-0.00639999889435816,1.33725589406987E-10,
2.62934110861178E-19));
#9503=CARTESIAN_POINT('Origin',(0.0075,-1.3010426069826E-19,1.1666015375944E-18));
#9504=CARTESIAN_POINT('',(0.00750000021337695,-1.12844211802569E-18,0.00860000022986174));
#9505=CARTESIAN_POINT('',(0.00750000021337695,-9.55567354576375E-13,-0.00860000022983698));
#9506=CARTESIAN_POINT('Origin',(0.00750000021337695,1.20438122943562E-10,
-1.36910420000699E-19));
#9507=CARTESIAN_POINT('Origin',(0.00750000021337695,-1.20438123513651E-10,
2.9038238015475E-19));
#9508=CARTESIAN_POINT('Origin',(-0.0206375,0.,-2.49552314011156E-51));
#9509=CARTESIAN_POINT('',(0.00639999944717908,-3.41326938021997E-12,0.00749999987620436));
#9510=CARTESIAN_POINT('',(-0.0206375,-9.18485099360515E-19,0.0075));
#9511=CARTESIAN_POINT('',(0.00639999944670613,1.23481356905966E-13,-0.0074999998349392));
#9512=CARTESIAN_POINT('Origin',(0.0064,-1.93061231994698E-18,-5.55111512312578E-18));
#9513=CARTESIAN_POINT('Origin',(0.00639999889435815,1.33725588774518E-10,
-1.62015184442301E-19));
#9514=CARTESIAN_POINT('Origin',(0.00639999889435815,-1.33725589355705E-10,
3.07932432666985E-19));
#9515=CARTESIAN_POINT('Origin',(0.00639999889435815,-4.29128599184298E-13,
0.00860000107142785));
#9516=CARTESIAN_POINT('Origin',(0.00639999889435815,-4.2911240869608E-13,
-0.00860000107142785));
#9517=CARTESIAN_POINT('Origin',(0.00639999889435815,1.33725588774518E-10,
-1.62015184442301E-19));
#11037=UNCERTAINTY_MEASURE_WITH_UNIT(LENGTH_MEASURE(1.E-5),#11113,
'DISTANCE_ACCURACY_VALUE',
'Maximum model space distance between geometric entities at asserted c
onnectivities');
#11073=UNCERTAINTY_MEASURE_WITH_UNIT(LENGTH_MEASURE(1.E-5),#11113,
'DISTANCE_ACCURACY_VALUE',
'Maximum model space distance between geometric entities at asserted c
onnectivities');
#11076=(
GEOMETRIC_REPRESENTATION_CONTEXT(3)
GLOBAL_UNCERTAINTY_ASSIGNED_CONTEXT((#11037))
GLOBAL_UNIT_ASSIGNED_CONTEXT((#11113,#11114,#11115))
REPRESENTATION_CONTEXT('','3D')
);
#11112=(
GEOMETRIC_REPRESENTATION_CONTEXT(3)
GLOBAL_UNCERTAINTY_ASSIGNED_CONTEXT((#11073))
GLOBAL_UNIT_ASSIGNED_CONTEXT((#11113,#11114,#11115))
REPRESENTATION_CONTEXT('','3D')
);
#11113=(
LENGTH_UNIT()
NAMED_UNIT(*)
SI_UNIT($,.METRE.)
);
#11114=(
NAMED_UNIT(*)
PLANE_ANGLE_UNIT()
SI_UNIT($,.RADIAN.)
);
#11115=(
NAMED_UNIT(*)
SI_UNIT($,.STERADIAN.)
SOLID_ANGLE_UNIT()
);
#11118=SHAPE_DEFINITION_REPRESENTATION(#11156,#11231);
#11156=PRODUCT_DEFINITION_SHAPE('',$,#11270);
#11231=SHAPE_REPRESENTATION('',(#6461),#11076);
#11267=PRODUCT_DEFINITION_CONTEXT('part definition',#11383,'design');
#11270=PRODUCT_DEFINITION('Radial Ball Bearing 1',
'Radial Ball Bearing 1',#11308,#11267);
#11308=PRODUCT_DEFINITION_FORMATION('',$,#11387);
#11383=APPLICATION_CONTEXT(
'Core Data for Automotive Mechanical Design Process');
#11384=PRODUCT_CONTEXT('part definition',#11383,'mechanical');
#11387=PRODUCT('Radial Ball Bearing 1','Radial Ball Bearing 1',
'radial ball bearing_68_as_AS_ISO 15 RBB - 415 - 6,SI,NC,6_68__ DE    
10847',(#11384));
#11425=PRESENTATION_STYLE_ASSIGNMENT((#11429));
#11429=SURFACE_STYLE_USAGE(.BOTH.,#11433);
#11433=SURFACE_SIDE_STYLE('',(#11437));
#11437=SURFACE_STYLE_FILL_AREA(#11441);
#11441=FILL_AREA_STYLE('Opaque(255,242,232)',(#11445));
#11445=FILL_AREA_STYLE_COLOUR('Opaque(255,242,232)',#11449);
#11449=COLOUR_RGB('Opaque(255,242,232)',1.,0.949019607843137,0.909803921568627);
ENDSEC;
END-ISO-10303-21;
